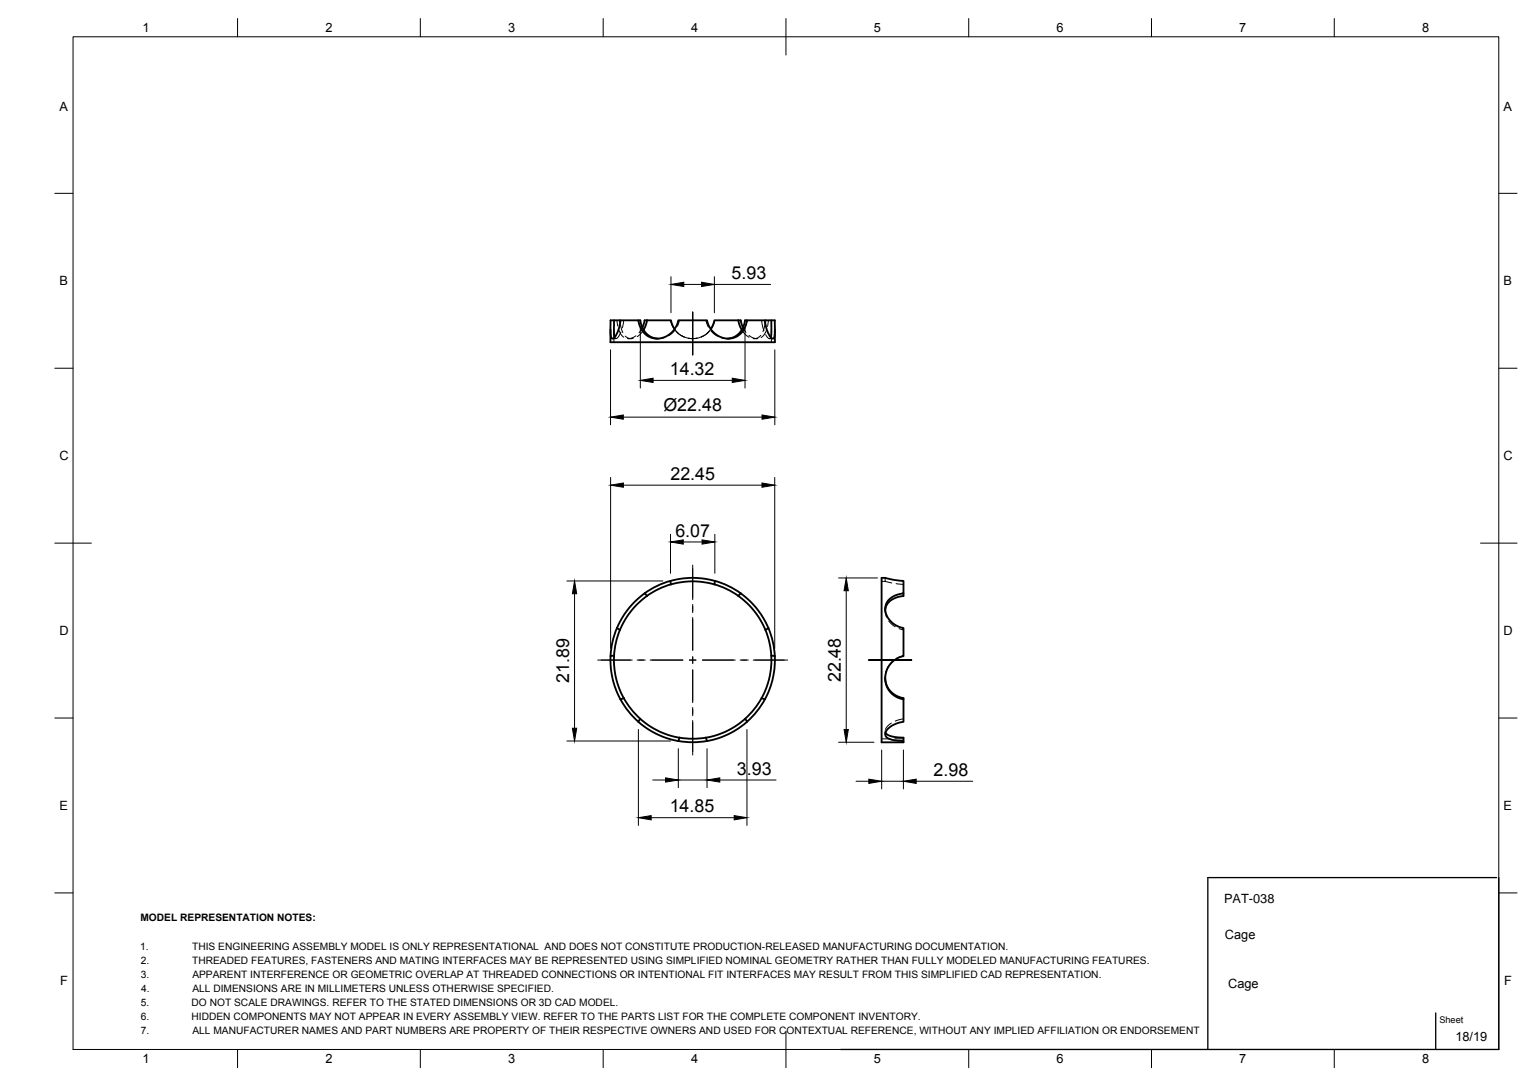
ISO-10303-21;
HEADER;
/* Generated by software containing ST-Developer
 * from STEP Tools, Inc. (www.steptools.com) 
 */

FILE_DESCRIPTION(
/* description */ ('Fork-mounted skate wheel'),
/* implementation_level */ '2;1');

FILE_NAME(
/* name */ 'Cage.step',
/* time_stamp */ '2026-10-29T16:11:26-07:00',
/* author */ (''),
/* organization */ (''),
/* preprocessor_version */ 'ST-DEVELOPER v20.2',
/* originating_system */ 'Autodesk Translation Framework v15.17.0.0',
/* authorisation */ '');

FILE_SCHEMA (('AUTOMOTIVE_DESIGN { 1 0 10303 214 3 1 1 }'));
ENDSEC;

DATA;
#10=MECHANICAL_DESIGN_GEOMETRIC_PRESENTATION_REPRESENTATION('',(#161),#3688);
#11=B_SPLINE_CURVE_WITH_KNOTS('',3,(#3211,#3212,#3213,#3214,#3215,#3216,
#3217,#3218,#3219,#3220,#3221,#3222,#3223,#3224,#3225,#3226,#3227,#3228,
#3229,#3230,#3231,#3232),.UNSPECIFIED.,.F.,.F.,(4,2,2,2,2,2,2,2,2,2,4),
(0.0591825211272536,0.157966726598481,0.236950089897721,0.315933453196962,
0.391576304923761,0.46721915665056,0.54286200837736,0.618504860104159,0.697488223403399,
0.77647158670264,0.875255792173867),.UNSPECIFIED.);
#12=B_SPLINE_CURVE_WITH_KNOTS('',3,(#3236,#3237,#3238,#3239,#3240,#3241,
#3242,#3243,#3244,#3245,#3246,#3247,#3248,#3249,#3250,#3251,#3252,#3253,
#3254,#3255,#3256,#3257),.UNSPECIFIED.,.F.,.F.,(4,2,2,2,2,2,2,2,2,2,4),
(0.0581119756758434,0.106553146291161,0.213106292582322,0.30849933801665,
0.386091982889075,0.4636846277615,0.541277272633925,0.61886991750635,0.714262962940678,
0.820816109231839,0.869257279847157),.UNSPECIFIED.);
#13=B_SPLINE_CURVE_WITH_KNOTS('',3,(#3263,#3264,#3265,#3266,#3267,#3268,
#3269,#3270,#3271,#3272,#3273,#3274,#3275,#3276,#3277,#3278,#3279,#3280,
#3281,#3282,#3283,#3284),.UNSPECIFIED.,.F.,.F.,(4,2,2,2,2,2,2,2,2,2,4),
(0.0581119756758434,0.106553146291161,0.213106292582322,0.30849933801665,
0.386091982889075,0.4636846277615,0.541277272633925,0.61886991750635,0.714262962940679,
0.820816109231839,0.869257279847157),.UNSPECIFIED.);
#14=B_SPLINE_CURVE_WITH_KNOTS('',3,(#3288,#3289,#3290,#3291,#3292,#3293,
#3294,#3295,#3296,#3297,#3298,#3299,#3300,#3301,#3302,#3303,#3304,#3305,
#3306,#3307,#3308,#3309),.UNSPECIFIED.,.F.,.F.,(4,2,2,2,2,2,2,2,2,2,4),
(0.0581119756758433,0.106553146291161,0.213106292582322,0.308499338016649,
0.386091982889075,0.4636846277615,0.541277272633925,0.61886991750635,0.714262962940678,
0.820816109231839,0.869257279847157),.UNSPECIFIED.);
#15=B_SPLINE_CURVE_WITH_KNOTS('',3,(#3318,#3319,#3320,#3321,#3322,#3323,
#3324,#3325,#3326,#3327,#3328,#3329,#3330,#3331,#3332,#3333,#3334,#3335,
#3336,#3337,#3338,#3339),.UNSPECIFIED.,.F.,.F.,(4,2,2,2,2,2,2,2,2,2,4),
(0.0581119756758433,0.106553146291161,0.213106292582322,0.30849933801665,
0.386091982889075,0.4636846277615,0.541277272633925,0.61886991750635,0.714262962940678,
0.820816109231839,0.869257279847157),.UNSPECIFIED.);
#16=B_SPLINE_CURVE_WITH_KNOTS('',3,(#3343,#3344,#3345,#3346,#3347,#3348,
#3349,#3350,#3351,#3352,#3353,#3354,#3355,#3356,#3357,#3358,#3359,#3360,
#3361,#3362,#3363,#3364),.UNSPECIFIED.,.F.,.F.,(4,2,2,2,2,2,2,2,2,2,4),
(0.0581119756758434,0.106553146291161,0.213106292582322,0.30849933801665,
0.386091982889075,0.4636846277615,0.541277272633925,0.61886991750635,0.714262962940678,
0.820816109231839,0.869257279847157),.UNSPECIFIED.);
#17=B_SPLINE_CURVE_WITH_KNOTS('',3,(#3368,#3369,#3370,#3371,#3372,#3373,
#3374,#3375,#3376,#3377,#3378,#3379,#3380,#3381,#3382,#3383,#3384,#3385,
#3386,#3387,#3388,#3389),.UNSPECIFIED.,.F.,.F.,(4,2,2,2,2,2,2,2,2,2,4),
(0.0581119756758434,0.106553146291161,0.213106292582322,0.30849933801665,
0.386091982889075,0.4636846277615,0.541277272633925,0.61886991750635,0.714262962940678,
0.820816109231839,0.869257279847157),.UNSPECIFIED.);
#18=B_SPLINE_CURVE_WITH_KNOTS('',3,(#3393,#3394,#3395,#3396,#3397,#3398,
#3399,#3400,#3401,#3402,#3403,#3404,#3405,#3406,#3407,#3408,#3409,#3410,
#3411,#3412,#3413,#3414),.UNSPECIFIED.,.F.,.F.,(4,2,2,2,2,2,2,2,2,2,4),
(0.0581119756758433,0.106553146291161,0.213106292582322,0.30849933801665,
0.386091982889075,0.4636846277615,0.541277272633925,0.61886991750635,0.714262962940678,
0.820816109231839,0.869257279847157),.UNSPECIFIED.);
#19=B_SPLINE_CURVE_WITH_KNOTS('',3,(#3422,#3423,#3424,#3425,#3426,#3427,
#3428,#3429,#3430,#3431,#3432,#3433,#3434,#3435,#3436,#3437,#3438,#3439,
#3440,#3441,#3442,#3443),.UNSPECIFIED.,.F.,.F.,(4,2,2,2,2,2,2,2,2,2,4),
(0.0591825211272536,0.157966726598481,0.236950089897721,0.315933453196962,
0.391576304923761,0.467219156650561,0.54286200837736,0.618504860104159,
0.697488223403399,0.77647158670264,0.875255792173867),.UNSPECIFIED.);
#20=B_SPLINE_CURVE_WITH_KNOTS('',3,(#3451,#3452,#3453,#3454,#3455,#3456,
#3457,#3458,#3459,#3460,#3461,#3462,#3463,#3464,#3465,#3466,#3467,#3468,
#3469,#3470,#3471,#3472),.UNSPECIFIED.,.F.,.F.,(4,2,2,2,2,2,2,2,2,2,4),
(0.0591825211272536,0.157966726598481,0.236950089897722,0.315933453196962,
0.391576304923761,0.467219156650561,0.54286200837736,0.618504860104159,
0.697488223403399,0.77647158670264,0.875255792173867),.UNSPECIFIED.);
#21=B_SPLINE_CURVE_WITH_KNOTS('',3,(#3482,#3483,#3484,#3485,#3486,#3487,
#3488,#3489,#3490,#3491,#3492,#3493,#3494,#3495,#3496,#3497,#3498,#3499,
#3500,#3501,#3502,#3503),.UNSPECIFIED.,.F.,.F.,(4,2,2,2,2,2,2,2,2,2,4),
(0.0591825211272536,0.157966726598481,0.236950089897721,0.315933453196962,
0.391576304923761,0.46721915665056,0.54286200837736,0.618504860104159,0.697488223403399,
0.77647158670264,0.875255792173867),.UNSPECIFIED.);
#22=B_SPLINE_CURVE_WITH_KNOTS('',3,(#3511,#3512,#3513,#3514,#3515,#3516,
#3517,#3518,#3519,#3520,#3521,#3522,#3523,#3524,#3525,#3526,#3527,#3528,
#3529,#3530,#3531,#3532),.UNSPECIFIED.,.F.,.F.,(4,2,2,2,2,2,2,2,2,2,4),
(0.0591825211272536,0.157966726598481,0.236950089897721,0.315933453196962,
0.391576304923761,0.46721915665056,0.542862008377359,0.618504860104159,
0.697488223403399,0.776471586702639,0.875255792173867),.UNSPECIFIED.);
#23=B_SPLINE_CURVE_WITH_KNOTS('',3,(#3540,#3541,#3542,#3543,#3544,#3545,
#3546,#3547,#3548,#3549,#3550,#3551,#3552,#3553,#3554,#3555,#3556,#3557,
#3558,#3559,#3560,#3561),.UNSPECIFIED.,.F.,.F.,(4,2,2,2,2,2,2,2,2,2,4),
(0.0591825211272536,0.157966726598481,0.236950089897721,0.315933453196962,
0.391576304923761,0.46721915665056,0.54286200837736,0.618504860104159,0.697488223403399,
0.77647158670264,0.875255792173867),.UNSPECIFIED.);
#24=B_SPLINE_CURVE_WITH_KNOTS('',3,(#3570,#3571,#3572,#3573,#3574,#3575,
#3576,#3577,#3578,#3579,#3580,#3581,#3582,#3583,#3584,#3585,#3586,#3587,
#3588,#3589,#3590,#3591),.UNSPECIFIED.,.F.,.F.,(4,2,2,2,2,2,2,2,2,2,4),
(0.0591825211272536,0.157966726598481,0.236950089897721,0.315933453196962,
0.391576304923761,0.46721915665056,0.542862008377359,0.618504860104159,
0.697488223403399,0.776471586702639,0.875255792173867),.UNSPECIFIED.);
#32=SPHERICAL_SURFACE('',#2134,0.309556);
#33=SPHERICAL_SURFACE('',#2150,0.309556);
#34=SPHERICAL_SURFACE('',#2155,0.309556);
#35=SPHERICAL_SURFACE('',#2161,0.309556);
#36=SPHERICAL_SURFACE('',#2166,0.309556);
#37=SPHERICAL_SURFACE('',#2171,0.309556);
#38=SPHERICAL_SURFACE('',#2179,0.309556);
#131=SHAPE_REPRESENTATION_RELATIONSHIP('SRR','None',#3756,#143);
#143=ADVANCED_BREP_SHAPE_REPRESENTATION('',(#179),#3685);
#161=STYLED_ITEM('',(#3896),#179);
#179=MANIFOLD_SOLID_BREP('Continuous crown cage',#1823);
#212=FACE_BOUND('',#518,.T.);
#262=PLANE('',#2147);
#263=PLANE('',#2152);
#264=PLANE('',#2157);
#265=PLANE('',#2163);
#266=PLANE('',#2168);
#267=PLANE('',#2177);
#268=PLANE('',#2181);
#269=PLANE('',#2182);
#360=FACE_OUTER_BOUND('',#502,.T.);
#361=FACE_OUTER_BOUND('',#503,.T.);
#362=FACE_OUTER_BOUND('',#504,.T.);
#363=FACE_OUTER_BOUND('',#505,.T.);
#364=FACE_OUTER_BOUND('',#506,.T.);
#365=FACE_OUTER_BOUND('',#507,.T.);
#366=FACE_OUTER_BOUND('',#508,.T.);
#367=FACE_OUTER_BOUND('',#509,.T.);
#368=FACE_OUTER_BOUND('',#510,.T.);
#369=FACE_OUTER_BOUND('',#511,.T.);
#370=FACE_OUTER_BOUND('',#512,.T.);
#371=FACE_OUTER_BOUND('',#513,.T.);
#372=FACE_OUTER_BOUND('',#514,.T.);
#373=FACE_OUTER_BOUND('',#515,.T.);
#374=FACE_OUTER_BOUND('',#516,.T.);
#375=FACE_OUTER_BOUND('',#517,.T.);
#376=FACE_OUTER_BOUND('',#519,.T.);
#502=EDGE_LOOP('',(#1529,#1530,#1531,#1532));
#503=EDGE_LOOP('',(#1533,#1534,#1535,#1536,#1537,#1538,#1539,#1540,#1541,
#1542,#1543,#1544,#1545,#1546,#1547,#1548,#1549,#1550));
#504=EDGE_LOOP('',(#1551,#1552,#1553,#1554));
#505=EDGE_LOOP('',(#1555,#1556,#1557,#1558));
#506=EDGE_LOOP('',(#1559,#1560,#1561,#1562));
#507=EDGE_LOOP('',(#1563,#1564,#1565,#1566));
#508=EDGE_LOOP('',(#1567,#1568,#1569,#1570,#1571,#1572));
#509=EDGE_LOOP('',(#1573,#1574,#1575,#1576));
#510=EDGE_LOOP('',(#1577,#1578,#1579,#1580));
#511=EDGE_LOOP('',(#1581,#1582,#1583,#1584));
#512=EDGE_LOOP('',(#1585,#1586,#1587,#1588));
#513=EDGE_LOOP('',(#1589,#1590,#1591,#1592));
#514=EDGE_LOOP('',(#1593,#1594,#1595,#1596,#1597,#1598,#1599,#1600,#1601,
#1602,#1603,#1604,#1605,#1606,#1607,#1608,#1609,#1610));
#515=EDGE_LOOP('',(#1611,#1612,#1613,#1614));
#516=EDGE_LOOP('',(#1615,#1616,#1617,#1618));
#517=EDGE_LOOP('',(#1619));
#518=EDGE_LOOP('',(#1620));
#519=EDGE_LOOP('',(#1621,#1622,#1623,#1624));
#624=LINE('',#3313,#718);
#625=LINE('',#3566,#719);
#718=VECTOR('',#2669,1.123812);
#719=VECTOR('',#2738,1.076188);
#796=CIRCLE('',#2135,0.303778037777585);
#797=CIRCLE('',#2136,0.303778037777585);
#798=CIRCLE('',#2138,1.123812);
#799=CIRCLE('',#2139,1.123812);
#800=CIRCLE('',#2140,1.123812);
#801=CIRCLE('',#2141,1.123812);
#802=CIRCLE('',#2142,1.123812);
#803=CIRCLE('',#2143,1.123812);
#804=CIRCLE('',#2144,1.123812);
#805=CIRCLE('',#2145,1.123812);
#806=CIRCLE('',#2146,1.123812);
#807=CIRCLE('',#2148,1.076188);
#808=CIRCLE('',#2149,0.303778037777585);
#809=CIRCLE('',#2151,0.303778037777585);
#810=CIRCLE('',#2153,1.076188);
#811=CIRCLE('',#2154,0.303778037777585);
#812=CIRCLE('',#2156,0.303778037777585);
#813=CIRCLE('',#2158,1.076188);
#814=CIRCLE('',#2159,1.076188);
#815=CIRCLE('',#2160,0.303778037777585);
#816=CIRCLE('',#2162,0.303778037777585);
#817=CIRCLE('',#2164,1.076188);
#818=CIRCLE('',#2165,0.303778037777585);
#819=CIRCLE('',#2167,0.303778037777585);
#820=CIRCLE('',#2169,1.076188);
#821=CIRCLE('',#2170,0.303778037777585);
#822=CIRCLE('',#2172,0.303778037777585);
#823=CIRCLE('',#2174,1.076188);
#824=CIRCLE('',#2175,1.076188);
#825=CIRCLE('',#2176,1.076188);
#826=CIRCLE('',#2178,0.303778037777585);
#827=CIRCLE('',#2180,0.303778037777585);
#951=VERTEX_POINT('',#3209);
#952=VERTEX_POINT('',#3210);
#953=VERTEX_POINT('',#3233);
#954=VERTEX_POINT('',#3235);
#955=VERTEX_POINT('',#3260);
#956=VERTEX_POINT('',#3262);
#957=VERTEX_POINT('',#3285);
#958=VERTEX_POINT('',#3287);
#959=VERTEX_POINT('',#3310);
#960=VERTEX_POINT('',#3312);
#961=VERTEX_POINT('',#3315);
#962=VERTEX_POINT('',#3317);
#963=VERTEX_POINT('',#3340);
#964=VERTEX_POINT('',#3342);
#965=VERTEX_POINT('',#3365);
#966=VERTEX_POINT('',#3367);
#967=VERTEX_POINT('',#3390);
#968=VERTEX_POINT('',#3392);
#969=VERTEX_POINT('',#3417);
#970=VERTEX_POINT('',#3421);
#971=VERTEX_POINT('',#3446);
#972=VERTEX_POINT('',#3450);
#973=VERTEX_POINT('',#3475);
#974=VERTEX_POINT('',#3477);
#975=VERTEX_POINT('',#3481);
#976=VERTEX_POINT('',#3506);
#977=VERTEX_POINT('',#3510);
#978=VERTEX_POINT('',#3535);
#979=VERTEX_POINT('',#3539);
#980=VERTEX_POINT('',#3564);
#981=VERTEX_POINT('',#3567);
#982=VERTEX_POINT('',#3569);
#1151=EDGE_CURVE('',#951,#952,#11,.T.);
#1152=EDGE_CURVE('',#953,#951,#796,.T.);
#1153=EDGE_CURVE('',#954,#953,#12,.T.);
#1154=EDGE_CURVE('',#952,#954,#797,.T.);
#1155=EDGE_CURVE('',#955,#953,#798,.T.);
#1156=EDGE_CURVE('',#955,#956,#13,.T.);
#1157=EDGE_CURVE('',#957,#956,#799,.T.);
#1158=EDGE_CURVE('',#957,#958,#14,.T.);
#1159=EDGE_CURVE('',#959,#958,#800,.T.);
#1160=EDGE_CURVE('',#959,#960,#624,.T.);
#1161=EDGE_CURVE('',#960,#960,#801,.T.);
#1162=EDGE_CURVE('',#961,#959,#802,.T.);
#1163=EDGE_CURVE('',#961,#962,#15,.T.);
#1164=EDGE_CURVE('',#963,#962,#803,.T.);
#1165=EDGE_CURVE('',#963,#964,#16,.T.);
#1166=EDGE_CURVE('',#965,#964,#804,.T.);
#1167=EDGE_CURVE('',#965,#966,#17,.T.);
#1168=EDGE_CURVE('',#967,#966,#805,.T.);
#1169=EDGE_CURVE('',#967,#968,#18,.T.);
#1170=EDGE_CURVE('',#954,#968,#806,.T.);
#1171=EDGE_CURVE('',#951,#969,#807,.T.);
#1172=EDGE_CURVE('',#969,#955,#808,.T.);
#1173=EDGE_CURVE('',#970,#969,#19,.T.);
#1174=EDGE_CURVE('',#956,#970,#809,.T.);
#1175=EDGE_CURVE('',#970,#971,#810,.T.);
#1176=EDGE_CURVE('',#971,#957,#811,.T.);
#1177=EDGE_CURVE('',#972,#971,#20,.T.);
#1178=EDGE_CURVE('',#958,#972,#812,.T.);
#1179=EDGE_CURVE('',#972,#973,#813,.T.);
#1180=EDGE_CURVE('',#973,#974,#814,.T.);
#1181=EDGE_CURVE('',#974,#961,#815,.T.);
#1182=EDGE_CURVE('',#975,#974,#21,.T.);
#1183=EDGE_CURVE('',#962,#975,#816,.T.);
#1184=EDGE_CURVE('',#975,#976,#817,.T.);
#1185=EDGE_CURVE('',#976,#963,#818,.T.);
#1186=EDGE_CURVE('',#977,#976,#22,.T.);
#1187=EDGE_CURVE('',#964,#977,#819,.T.);
#1188=EDGE_CURVE('',#977,#978,#820,.T.);
#1189=EDGE_CURVE('',#978,#965,#821,.T.);
#1190=EDGE_CURVE('',#979,#978,#23,.T.);
#1191=EDGE_CURVE('',#966,#979,#822,.T.);
#1192=EDGE_CURVE('',#980,#980,#823,.T.);
#1193=EDGE_CURVE('',#980,#973,#625,.T.);
#1194=EDGE_CURVE('',#981,#952,#824,.T.);
#1195=EDGE_CURVE('',#981,#982,#24,.T.);
#1196=EDGE_CURVE('',#979,#982,#825,.T.);
#1197=EDGE_CURVE('',#968,#981,#826,.T.);
#1198=EDGE_CURVE('',#982,#967,#827,.T.);
#1529=ORIENTED_EDGE('',*,*,#1151,.F.);
#1530=ORIENTED_EDGE('',*,*,#1152,.F.);
#1531=ORIENTED_EDGE('',*,*,#1153,.F.);
#1532=ORIENTED_EDGE('',*,*,#1154,.F.);
#1533=ORIENTED_EDGE('',*,*,#1153,.T.);
#1534=ORIENTED_EDGE('',*,*,#1155,.F.);
#1535=ORIENTED_EDGE('',*,*,#1156,.T.);
#1536=ORIENTED_EDGE('',*,*,#1157,.F.);
#1537=ORIENTED_EDGE('',*,*,#1158,.T.);
#1538=ORIENTED_EDGE('',*,*,#1159,.F.);
#1539=ORIENTED_EDGE('',*,*,#1160,.T.);
#1540=ORIENTED_EDGE('',*,*,#1161,.F.);
#1541=ORIENTED_EDGE('',*,*,#1160,.F.);
#1542=ORIENTED_EDGE('',*,*,#1162,.F.);
#1543=ORIENTED_EDGE('',*,*,#1163,.T.);
#1544=ORIENTED_EDGE('',*,*,#1164,.F.);
#1545=ORIENTED_EDGE('',*,*,#1165,.T.);
#1546=ORIENTED_EDGE('',*,*,#1166,.F.);
#1547=ORIENTED_EDGE('',*,*,#1167,.T.);
#1548=ORIENTED_EDGE('',*,*,#1168,.F.);
#1549=ORIENTED_EDGE('',*,*,#1169,.T.);
#1550=ORIENTED_EDGE('',*,*,#1170,.F.);
#1551=ORIENTED_EDGE('',*,*,#1152,.T.);
#1552=ORIENTED_EDGE('',*,*,#1171,.T.);
#1553=ORIENTED_EDGE('',*,*,#1172,.T.);
#1554=ORIENTED_EDGE('',*,*,#1155,.T.);
#1555=ORIENTED_EDGE('',*,*,#1173,.F.);
#1556=ORIENTED_EDGE('',*,*,#1174,.F.);
#1557=ORIENTED_EDGE('',*,*,#1156,.F.);
#1558=ORIENTED_EDGE('',*,*,#1172,.F.);
#1559=ORIENTED_EDGE('',*,*,#1174,.T.);
#1560=ORIENTED_EDGE('',*,*,#1175,.T.);
#1561=ORIENTED_EDGE('',*,*,#1176,.T.);
#1562=ORIENTED_EDGE('',*,*,#1157,.T.);
#1563=ORIENTED_EDGE('',*,*,#1177,.F.);
#1564=ORIENTED_EDGE('',*,*,#1178,.F.);
#1565=ORIENTED_EDGE('',*,*,#1158,.F.);
#1566=ORIENTED_EDGE('',*,*,#1176,.F.);
#1567=ORIENTED_EDGE('',*,*,#1178,.T.);
#1568=ORIENTED_EDGE('',*,*,#1179,.T.);
#1569=ORIENTED_EDGE('',*,*,#1180,.T.);
#1570=ORIENTED_EDGE('',*,*,#1181,.T.);
#1571=ORIENTED_EDGE('',*,*,#1162,.T.);
#1572=ORIENTED_EDGE('',*,*,#1159,.T.);
#1573=ORIENTED_EDGE('',*,*,#1182,.F.);
#1574=ORIENTED_EDGE('',*,*,#1183,.F.);
#1575=ORIENTED_EDGE('',*,*,#1163,.F.);
#1576=ORIENTED_EDGE('',*,*,#1181,.F.);
#1577=ORIENTED_EDGE('',*,*,#1183,.T.);
#1578=ORIENTED_EDGE('',*,*,#1184,.T.);
#1579=ORIENTED_EDGE('',*,*,#1185,.T.);
#1580=ORIENTED_EDGE('',*,*,#1164,.T.);
#1581=ORIENTED_EDGE('',*,*,#1186,.F.);
#1582=ORIENTED_EDGE('',*,*,#1187,.F.);
#1583=ORIENTED_EDGE('',*,*,#1165,.F.);
#1584=ORIENTED_EDGE('',*,*,#1185,.F.);
#1585=ORIENTED_EDGE('',*,*,#1187,.T.);
#1586=ORIENTED_EDGE('',*,*,#1188,.T.);
#1587=ORIENTED_EDGE('',*,*,#1189,.T.);
#1588=ORIENTED_EDGE('',*,*,#1166,.T.);
#1589=ORIENTED_EDGE('',*,*,#1167,.F.);
#1590=ORIENTED_EDGE('',*,*,#1189,.F.);
#1591=ORIENTED_EDGE('',*,*,#1190,.F.);
#1592=ORIENTED_EDGE('',*,*,#1191,.F.);
#1593=ORIENTED_EDGE('',*,*,#1192,.F.);
#1594=ORIENTED_EDGE('',*,*,#1193,.T.);
#1595=ORIENTED_EDGE('',*,*,#1179,.F.);
#1596=ORIENTED_EDGE('',*,*,#1177,.T.);
#1597=ORIENTED_EDGE('',*,*,#1175,.F.);
#1598=ORIENTED_EDGE('',*,*,#1173,.T.);
#1599=ORIENTED_EDGE('',*,*,#1171,.F.);
#1600=ORIENTED_EDGE('',*,*,#1151,.T.);
#1601=ORIENTED_EDGE('',*,*,#1194,.F.);
#1602=ORIENTED_EDGE('',*,*,#1195,.T.);
#1603=ORIENTED_EDGE('',*,*,#1196,.F.);
#1604=ORIENTED_EDGE('',*,*,#1190,.T.);
#1605=ORIENTED_EDGE('',*,*,#1188,.F.);
#1606=ORIENTED_EDGE('',*,*,#1186,.T.);
#1607=ORIENTED_EDGE('',*,*,#1184,.F.);
#1608=ORIENTED_EDGE('',*,*,#1182,.T.);
#1609=ORIENTED_EDGE('',*,*,#1180,.F.);
#1610=ORIENTED_EDGE('',*,*,#1193,.F.);
#1611=ORIENTED_EDGE('',*,*,#1154,.T.);
#1612=ORIENTED_EDGE('',*,*,#1170,.T.);
#1613=ORIENTED_EDGE('',*,*,#1197,.T.);
#1614=ORIENTED_EDGE('',*,*,#1194,.T.);
#1615=ORIENTED_EDGE('',*,*,#1169,.F.);
#1616=ORIENTED_EDGE('',*,*,#1198,.F.);
#1617=ORIENTED_EDGE('',*,*,#1195,.F.);
#1618=ORIENTED_EDGE('',*,*,#1197,.F.);
#1619=ORIENTED_EDGE('',*,*,#1161,.T.);
#1620=ORIENTED_EDGE('',*,*,#1192,.T.);
#1621=ORIENTED_EDGE('',*,*,#1191,.T.);
#1622=ORIENTED_EDGE('',*,*,#1196,.T.);
#1623=ORIENTED_EDGE('',*,*,#1198,.T.);
#1624=ORIENTED_EDGE('',*,*,#1168,.T.);
#1686=CYLINDRICAL_SURFACE('',#2137,1.123812);
#1687=CYLINDRICAL_SURFACE('',#2173,1.076188);
#1778=ADVANCED_FACE('',(#360),#32,.F.);
#1779=ADVANCED_FACE('',(#361),#1686,.T.);
#1780=ADVANCED_FACE('',(#362),#262,.T.);
#1781=ADVANCED_FACE('',(#363),#33,.F.);
#1782=ADVANCED_FACE('',(#364),#263,.T.);
#1783=ADVANCED_FACE('',(#365),#34,.F.);
#1784=ADVANCED_FACE('',(#366),#264,.T.);
#1785=ADVANCED_FACE('',(#367),#35,.F.);
#1786=ADVANCED_FACE('',(#368),#265,.T.);
#1787=ADVANCED_FACE('',(#369),#36,.F.);
#1788=ADVANCED_FACE('',(#370),#266,.T.);
#1789=ADVANCED_FACE('',(#371),#37,.F.);
#1790=ADVANCED_FACE('',(#372),#1687,.F.);
#1791=ADVANCED_FACE('',(#373),#267,.T.);
#1792=ADVANCED_FACE('',(#374),#38,.F.);
#1793=ADVANCED_FACE('',(#375,#212),#268,.T.);
#1794=ADVANCED_FACE('',(#376),#269,.T.);
#1823=CLOSED_SHELL('',(#1778,#1779,#1780,#1781,#1782,#1783,#1784,#1785,
#1786,#1787,#1788,#1789,#1790,#1791,#1792,#1793,#1794));
#2133=AXIS2_PLACEMENT_3D('',#3207,#2653,#2654);
#2134=AXIS2_PLACEMENT_3D('',#3208,#2655,#2656);
#2135=AXIS2_PLACEMENT_3D('',#3234,#2657,#2658);
#2136=AXIS2_PLACEMENT_3D('',#3258,#2659,#2660);
#2137=AXIS2_PLACEMENT_3D('',#3259,#2661,#2662);
#2138=AXIS2_PLACEMENT_3D('',#3261,#2663,#2664);
#2139=AXIS2_PLACEMENT_3D('',#3286,#2665,#2666);
#2140=AXIS2_PLACEMENT_3D('',#3311,#2667,#2668);
#2141=AXIS2_PLACEMENT_3D('',#3314,#2670,#2671);
#2142=AXIS2_PLACEMENT_3D('',#3316,#2672,#2673);
#2143=AXIS2_PLACEMENT_3D('',#3341,#2674,#2675);
#2144=AXIS2_PLACEMENT_3D('',#3366,#2676,#2677);
#2145=AXIS2_PLACEMENT_3D('',#3391,#2678,#2679);
#2146=AXIS2_PLACEMENT_3D('',#3415,#2680,#2681);
#2147=AXIS2_PLACEMENT_3D('',#3416,#2682,#2683);
#2148=AXIS2_PLACEMENT_3D('',#3418,#2684,#2685);
#2149=AXIS2_PLACEMENT_3D('',#3419,#2686,#2687);
#2150=AXIS2_PLACEMENT_3D('',#3420,#2688,#2689);
#2151=AXIS2_PLACEMENT_3D('',#3444,#2690,#2691);
#2152=AXIS2_PLACEMENT_3D('',#3445,#2692,#2693);
#2153=AXIS2_PLACEMENT_3D('',#3447,#2694,#2695);
#2154=AXIS2_PLACEMENT_3D('',#3448,#2696,#2697);
#2155=AXIS2_PLACEMENT_3D('',#3449,#2698,#2699);
#2156=AXIS2_PLACEMENT_3D('',#3473,#2700,#2701);
#2157=AXIS2_PLACEMENT_3D('',#3474,#2702,#2703);
#2158=AXIS2_PLACEMENT_3D('',#3476,#2704,#2705);
#2159=AXIS2_PLACEMENT_3D('',#3478,#2706,#2707);
#2160=AXIS2_PLACEMENT_3D('',#3479,#2708,#2709);
#2161=AXIS2_PLACEMENT_3D('',#3480,#2710,#2711);
#2162=AXIS2_PLACEMENT_3D('',#3504,#2712,#2713);
#2163=AXIS2_PLACEMENT_3D('',#3505,#2714,#2715);
#2164=AXIS2_PLACEMENT_3D('',#3507,#2716,#2717);
#2165=AXIS2_PLACEMENT_3D('',#3508,#2718,#2719);
#2166=AXIS2_PLACEMENT_3D('',#3509,#2720,#2721);
#2167=AXIS2_PLACEMENT_3D('',#3533,#2722,#2723);
#2168=AXIS2_PLACEMENT_3D('',#3534,#2724,#2725);
#2169=AXIS2_PLACEMENT_3D('',#3536,#2726,#2727);
#2170=AXIS2_PLACEMENT_3D('',#3537,#2728,#2729);
#2171=AXIS2_PLACEMENT_3D('',#3538,#2730,#2731);
#2172=AXIS2_PLACEMENT_3D('',#3562,#2732,#2733);
#2173=AXIS2_PLACEMENT_3D('',#3563,#2734,#2735);
#2174=AXIS2_PLACEMENT_3D('',#3565,#2736,#2737);
#2175=AXIS2_PLACEMENT_3D('',#3568,#2739,#2740);
#2176=AXIS2_PLACEMENT_3D('',#3592,#2741,#2742);
#2177=AXIS2_PLACEMENT_3D('',#3593,#2743,#2744);
#2178=AXIS2_PLACEMENT_3D('',#3594,#2745,#2746);
#2179=AXIS2_PLACEMENT_3D('',#3595,#2747,#2748);
#2180=AXIS2_PLACEMENT_3D('',#3596,#2749,#2750);
#2181=AXIS2_PLACEMENT_3D('',#3597,#2751,#2752);
#2182=AXIS2_PLACEMENT_3D('',#3598,#2753,#2754);
#2653=DIRECTION('axis',(0.,0.,1.));
#2654=DIRECTION('refdir',(1.,0.,0.));
#2655=DIRECTION('center_axis',(0.,0.,1.));
#2656=DIRECTION('ref_axis',(1.,0.,0.));
#2657=DIRECTION('center_axis',(0.,-1.,0.));
#2658=DIRECTION('ref_axis',(0.,0.,-1.));
#2659=DIRECTION('center_axis',(0.,-1.,0.));
#2660=DIRECTION('ref_axis',(0.,0.,-1.));
#2661=DIRECTION('center_axis',(0.,1.,0.));
#2662=DIRECTION('ref_axis',(1.,0.,0.));
#2663=DIRECTION('center_axis',(0.,1.,0.));
#2664=DIRECTION('ref_axis',(1.,0.,0.));
#2665=DIRECTION('center_axis',(0.,1.,0.));
#2666=DIRECTION('ref_axis',(1.,0.,0.));
#2667=DIRECTION('center_axis',(0.,1.,0.));
#2668=DIRECTION('ref_axis',(1.,0.,0.));
#2669=DIRECTION('',(0.,-1.,0.));
#2670=DIRECTION('center_axis',(0.,-1.,0.));
#2671=DIRECTION('ref_axis',(1.,0.,0.));
#2672=DIRECTION('center_axis',(0.,1.,0.));
#2673=DIRECTION('ref_axis',(1.,0.,0.));
#2674=DIRECTION('center_axis',(0.,1.,0.));
#2675=DIRECTION('ref_axis',(1.,0.,0.));
#2676=DIRECTION('center_axis',(0.,1.,0.));
#2677=DIRECTION('ref_axis',(1.,0.,0.));
#2678=DIRECTION('center_axis',(0.,1.,0.));
#2679=DIRECTION('ref_axis',(1.,0.,0.));
#2680=DIRECTION('center_axis',(0.,1.,0.));
#2681=DIRECTION('ref_axis',(1.,0.,0.));
#2682=DIRECTION('center_axis',(0.,1.,0.));
#2683=DIRECTION('ref_axis',(1.,0.,0.));
#2684=DIRECTION('center_axis',(0.,-1.,0.));
#2685=DIRECTION('ref_axis',(1.,0.,0.));
#2686=DIRECTION('center_axis',(0.,-1.,0.));
#2687=DIRECTION('ref_axis',(0.,0.,-1.));
#2688=DIRECTION('center_axis',(8.96625347776458E-17,0.,1.));
#2689=DIRECTION('ref_axis',(1.,0.,0.));
#2690=DIRECTION('center_axis',(0.,-1.,0.));
#2691=DIRECTION('ref_axis',(0.,0.,-1.));
#2692=DIRECTION('center_axis',(0.,1.,0.));
#2693=DIRECTION('ref_axis',(1.,0.,0.));
#2694=DIRECTION('center_axis',(0.,-1.,0.));
#2695=DIRECTION('ref_axis',(1.,0.,0.));
#2696=DIRECTION('center_axis',(0.,-1.,0.));
#2697=DIRECTION('ref_axis',(0.,0.,-1.));
#2698=DIRECTION('center_axis',(0.,0.,1.));
#2699=DIRECTION('ref_axis',(1.,0.,0.));
#2700=DIRECTION('center_axis',(0.,-1.,0.));
#2701=DIRECTION('ref_axis',(0.,0.,-1.));
#2702=DIRECTION('center_axis',(0.,1.,0.));
#2703=DIRECTION('ref_axis',(1.,0.,0.));
#2704=DIRECTION('center_axis',(0.,-1.,0.));
#2705=DIRECTION('ref_axis',(1.,0.,0.));
#2706=DIRECTION('center_axis',(0.,-1.,0.));
#2707=DIRECTION('ref_axis',(1.,0.,0.));
#2708=DIRECTION('center_axis',(0.,-1.,0.));
#2709=DIRECTION('ref_axis',(0.,0.,-1.));
#2710=DIRECTION('center_axis',(0.,0.,1.));
#2711=DIRECTION('ref_axis',(1.,0.,0.));
#2712=DIRECTION('center_axis',(0.,-1.,0.));
#2713=DIRECTION('ref_axis',(0.,0.,-1.));
#2714=DIRECTION('center_axis',(0.,1.,0.));
#2715=DIRECTION('ref_axis',(1.,0.,0.));
#2716=DIRECTION('center_axis',(0.,-1.,0.));
#2717=DIRECTION('ref_axis',(1.,0.,0.));
#2718=DIRECTION('center_axis',(0.,-1.,0.));
#2719=DIRECTION('ref_axis',(0.,0.,-1.));
#2720=DIRECTION('center_axis',(8.96625347776458E-17,0.,1.));
#2721=DIRECTION('ref_axis',(1.,0.,0.));
#2722=DIRECTION('center_axis',(0.,-1.,0.));
#2723=DIRECTION('ref_axis',(0.,0.,-1.));
#2724=DIRECTION('center_axis',(0.,1.,0.));
#2725=DIRECTION('ref_axis',(1.,0.,0.));
#2726=DIRECTION('center_axis',(0.,-1.,0.));
#2727=DIRECTION('ref_axis',(1.,0.,0.));
#2728=DIRECTION('center_axis',(0.,-1.,0.));
#2729=DIRECTION('ref_axis',(0.,0.,-1.));
#2730=DIRECTION('center_axis',(0.,0.,1.));
#2731=DIRECTION('ref_axis',(1.,0.,0.));
#2732=DIRECTION('center_axis',(0.,-1.,0.));
#2733=DIRECTION('ref_axis',(0.,0.,-1.));
#2734=DIRECTION('center_axis',(0.,1.,0.));
#2735=DIRECTION('ref_axis',(1.,0.,0.));
#2736=DIRECTION('center_axis',(0.,1.,0.));
#2737=DIRECTION('ref_axis',(1.,0.,0.));
#2738=DIRECTION('',(0.,1.,0.));
#2739=DIRECTION('center_axis',(0.,-1.,0.));
#2740=DIRECTION('ref_axis',(1.,0.,0.));
#2741=DIRECTION('center_axis',(0.,-1.,0.));
#2742=DIRECTION('ref_axis',(1.,0.,0.));
#2743=DIRECTION('center_axis',(0.,1.,0.));
#2744=DIRECTION('ref_axis',(1.,0.,0.));
#2745=DIRECTION('center_axis',(0.,-1.,0.));
#2746=DIRECTION('ref_axis',(0.,0.,-1.));
#2747=DIRECTION('center_axis',(0.,0.,1.));
#2748=DIRECTION('ref_axis',(1.,0.,0.));
#2749=DIRECTION('center_axis',(0.,-1.,0.));
#2750=DIRECTION('ref_axis',(0.,0.,-1.));
#2751=DIRECTION('center_axis',(0.,-1.,0.));
#2752=DIRECTION('ref_axis',(-1.,0.,0.));
#2753=DIRECTION('center_axis',(0.,1.,0.));
#2754=DIRECTION('ref_axis',(1.,0.,0.));
#3207=CARTESIAN_POINT('',(0.,0.,0.));
#3208=CARTESIAN_POINT('Origin',(0.685838782044607,0.,0.860014630714833));
#3209=CARTESIAN_POINT('',(0.413083465285518,-0.05953,0.993751811093549));
#3210=CARTESIAN_POINT('',(0.876916659919095,-0.05953,0.623857181492959));
#3211=CARTESIAN_POINT('Ctrl Pts',(0.413083465285518,-0.05953,0.993751811093549));
#3212=CARTESIAN_POINT('Ctrl Pts',(0.419070565453383,-0.0925528133349865,
0.991263089003441));
#3213=CARTESIAN_POINT('Ctrl Pts',(0.430199341854858,-0.124911173756694,
0.986608710139579));
#3214=CARTESIAN_POINT('Ctrl Pts',(0.457978755888596,-0.177924977804098,
0.973971221090534));
#3215=CARTESIAN_POINT('Ctrl Pts',(0.473077587363685,-0.199697230012983,
0.966820759530997));
#3216=CARTESIAN_POINT('Ctrl Pts',(0.507057380724533,-0.237895043532788,
0.949440676105255));
#3217=CARTESIAN_POINT('Ctrl Pts',(0.525933334162555,-0.254319232363049,
0.939198248544428));
#3218=CARTESIAN_POINT('Ctrl Pts',(0.564362943424238,-0.28018331644634,0.916597376014514));
#3219=CARTESIAN_POINT('Ctrl Pts',(0.585840553788742,-0.29104845371857,0.903141581680914));
#3220=CARTESIAN_POINT('Ctrl Pts',(0.629305439856167,-0.30527573347708,0.873412008702649));
#3221=CARTESIAN_POINT('Ctrl Pts',(0.651278921914856,-0.308638795020976,
0.857118508332695));
#3222=CARTESIAN_POINT('Ctrl Pts',(0.690705563850638,-0.308638795020976,
0.825676810575914));
#3223=CARTESIAN_POINT('Ctrl Pts',(0.711480111898423,-0.30527573347708,0.807879894508811));
#3224=CARTESIAN_POINT('Ctrl Pts',(0.750136149454208,-0.29104845371857,0.772120216227122));
#3225=CARTESIAN_POINT('Ctrl Pts',(0.768033796848072,-0.28018331644634,0.754175290318038));
#3226=CARTESIAN_POINT('Ctrl Pts',(0.798619410861634,-0.254319232363049,
0.721738358858166));
#3227=CARTESIAN_POINT('Ctrl Pts',(0.812805334167529,-0.237895043532788,
0.705614819529209));
#3228=CARTESIAN_POINT('Ctrl Pts',(0.837310877969633,-0.199697230012983,
0.676354402927683));
#3229=CARTESIAN_POINT('Ctrl Pts',(0.847641868610495,-0.177924977804098,
0.663225258065736));
#3230=CARTESIAN_POINT('Ctrl Pts',(0.866144010579847,-0.124911173756694,
0.638954437806245));
#3231=CARTESIAN_POINT('Ctrl Pts',(0.873158080166742,-0.0925528133349865,
0.62914037979579));
#3232=CARTESIAN_POINT('Ctrl Pts',(0.876916659919095,-0.05953,0.623857181492959));
#3233=CARTESIAN_POINT('',(0.437601487681057,-0.05953,1.03511272300331));
#3234=CARTESIAN_POINT('Origin',(0.685838782044607,-0.05953,0.860014630714833));
#3235=CARTESIAN_POINT('',(0.911784794170997,-0.05953,0.656964154625313));
#3236=CARTESIAN_POINT('Ctrl Pts',(0.911784794170998,-0.0595300000000001,
0.656964154625312));
#3237=CARTESIAN_POINT('Ctrl Pts',(0.909827729890942,-0.0762225747374255,
0.659680317203144));
#3238=CARTESIAN_POINT('Ctrl Pts',(0.907004864562642,-0.0928409665394228,
0.663576540841106));
#3239=CARTESIAN_POINT('Ctrl Pts',(0.895234408667242,-0.144299303100741,
0.679480524217551));
#3240=CARTESIAN_POINT('Ctrl Pts',(0.882797231409153,-0.177024326825049,
0.695831250979106));
#3241=CARTESIAN_POINT('Ctrl Pts',(0.854332839576145,-0.227269801620064,
0.73042219438957));
#3242=CARTESIAN_POINT('Ctrl Pts',(0.834863020612702,-0.251265615809407,
0.752807465209441));
#3243=CARTESIAN_POINT('Ctrl Pts',(0.800439809856111,-0.279889827963178,
0.789147407129766));
#3244=CARTESIAN_POINT('Ctrl Pts',(0.781998747691871,-0.290879136862659,
0.80756613568454));
#3245=CARTESIAN_POINT('Ctrl Pts',(0.742239891936898,-0.305251990234487,
0.844254137480382));
#3246=CARTESIAN_POINT('Ctrl Pts',(0.720906778729541,-0.308638795020976,
0.862505527716294));
#3247=CARTESIAN_POINT('Ctrl Pts',(0.680463863683392,-0.308638795020976,
0.894757676234429));
#3248=CARTESIAN_POINT('Ctrl Pts',(0.657923009631182,-0.305251990234488,
0.91149460735272));
#3249=CARTESIAN_POINT('Ctrl Pts',(0.613307674922609,-0.290879136862659,
0.942092777160053));
#3250=CARTESIAN_POINT('Ctrl Pts',(0.591247219971725,-0.279889827963178,
0.955972930713954));
#3251=CARTESIAN_POINT('Ctrl Pts',(0.548158511259202,-0.251265615809407,
0.981446681891443));
#3252=CARTESIAN_POINT('Ctrl Pts',(0.522002043615455,-0.227269801620063,
0.995447160474328));
#3253=CARTESIAN_POINT('Ctrl Pts',(0.481944444320713,-0.177024326825049,
1.01550068154148));
#3254=CARTESIAN_POINT('Ctrl Pts',(0.463236132117164,-0.14429930310074,1.0239876538093));
#3255=CARTESIAN_POINT('Ctrl Pts',(0.445111721969657,-0.0928409665394226,
1.03192403056628));
#3256=CARTESIAN_POINT('Ctrl Pts',(0.440685038163619,-0.0762225747374254,
1.03380912944435));
#3257=CARTESIAN_POINT('Ctrl Pts',(0.437601487681056,-0.05953,1.03511272300331));
#3258=CARTESIAN_POINT('Origin',(0.685838782044607,-0.05953,0.860014630714833));
#3259=CARTESIAN_POINT('Origin',(0.,-0.208355,0.));
#3260=CARTESIAN_POINT('',(0.0548532617164168,-0.05953,1.12247250791415));
#3261=CARTESIAN_POINT('Origin',(0.,-0.05953,0.));
#3262=CARTESIAN_POINT('',(-0.536443649899848,-0.05953,0.987512846410683));
#3263=CARTESIAN_POINT('Ctrl Pts',(0.0548532617164173,-0.0595300000000001,
1.12247250791414));
#3264=CARTESIAN_POINT('Ctrl Pts',(0.05150947068137,-0.0762225747374254,
1.12263591311425));
#3265=CARTESIAN_POINT('Ctrl Pts',(0.0467032526342597,-0.0928409665394227,
1.12285816383385));
#3266=CARTESIAN_POINT('Ctrl Pts',(0.0269302585198975,-0.144299303100741,
1.12357162229597));
#3267=CARTESIAN_POINT('Ctrl Pts',(0.006392292392153,-0.177024326825049,
1.12404235695137));
#3268=CARTESIAN_POINT('Ctrl Pts',(-0.0383992541984087,-0.227269801620063,
1.12335509974011));
#3269=CARTESIAN_POINT('Ctrl Pts',(-0.0680399972366993,-0.251265615809407,
1.12208997038458));
#3270=CARTESIAN_POINT('Ctrl Pts',(-0.117914228755037,-0.279889827963178,
1.1178344036749));
#3271=CARTESIAN_POINT('Ctrl Pts',(-0.14381238480104,-0.290879136862659,
1.11490049012186));
#3272=CARTESIAN_POINT('Ctrl Pts',(-0.19728546073067,-0.305251990234488,
1.10669035995599));
#3273=CARTESIAN_POINT('Ctrl Pts',(-0.224855950742601,-0.308638795020976,
1.10139101611326));
#3274=CARTESIAN_POINT('Ctrl Pts',(-0.275287440920027,-0.308638795020976,
1.0898803575765));
#3275=CARTESIAN_POINT('Ctrl Pts',(-0.302426893214945,-0.305251990234488,
1.08269251410343));
#3276=CARTESIAN_POINT('Ctrl Pts',(-0.35416671187353,-0.290879136862659,
1.06688848765783));
#3277=CARTESIAN_POINT('Ctrl Pts',(-0.3787731215897,-0.279889827963178,1.05829506364875));
#3278=CARTESIAN_POINT('Ctrl Pts',(-0.425554672694338,-0.251265615809407,
1.04048957871266));
#3279=CARTESIAN_POINT('Ctrl Pts',(-0.452808978448581,-0.227269801620063,
1.02876878445619));
#3280=CARTESIAN_POINT('Ctrl Pts',(-0.493462957200432,-0.177024326825049,
1.0099536580922));
#3281=CARTESIAN_POINT('Ctrl Pts',(-0.511762781179148,-0.14429930310074,
1.00061845128527));
#3282=CARTESIAN_POINT('Ctrl Pts',(-0.529268075276157,-0.0928409665394226,
0.991396466802468));
#3283=CARTESIAN_POINT('Ctrl Pts',(-0.533501897135713,-0.0762225747374254,
0.989110885965947));
#3284=CARTESIAN_POINT('Ctrl Pts',(-0.536443649899848,-0.0595300000000001,
0.987512846410683));
#3285=CARTESIAN_POINT('',(-0.843383895613249,-0.05953,0.742736168477219));
#3286=CARTESIAN_POINT('Origin',(0.,-0.05953,0.));
#3287=CARTESIAN_POINT('',(-1.10653577764992,-0.05953,0.196295654879792));
#3288=CARTESIAN_POINT('Ctrl Pts',(-0.843383895613249,-0.0595300000000001,
0.742736168477219));
#3289=CARTESIAN_POINT('Ctrl Pts',(-0.84559647055299,-0.0762225747374255,
0.740223768851062));
#3290=CARTESIAN_POINT('Ctrl Pts',(-0.848766861100456,-0.0928409665394227,
0.736604687327351));
#3291=CARTESIAN_POINT('Ctrl Pts',(-0.861652925570091,-0.144299303100741,
0.721590372101268));
#3292=CARTESIAN_POINT('Ctrl Pts',(-0.87482617317514,-0.177024326825049,
0.705826641853758));
#3293=CARTESIAN_POINT('Ctrl Pts',(-0.902215926359523,-0.227269801620063,
0.670378702718353));
#3294=CARTESIAN_POINT('Ctrl Pts',(-0.919707509403859,-0.251265615809407,
0.646415841396062));
#3295=CARTESIAN_POINT('Ctrl Pts',(-0.947476448101718,-0.279889827963178,
0.604769294586516));
#3296=CARTESIAN_POINT('Ctrl Pts',(-0.961329858300736,-0.290879136862659,
0.582692035672022));
#3297=CARTESIAN_POINT('Ctrl Pts',(-0.988250837578047,-0.305251990234488,
0.535766169015486));
#3298=CARTESIAN_POINT('Ctrl Pts',(-1.00129756308006,-0.308638795020976,
0.510906605094603));
#3299=CARTESIAN_POINT('Ctrl Pts',(-1.02374168767024,-0.308638795020976,
0.46430090015576));
#3300=CARTESIAN_POINT('Ctrl Pts',(-1.03504317708586,-0.305251990234488,
0.438600874831839));
#3301=CARTESIAN_POINT('Ctrl Pts',(-1.05494634094458,-0.290879136862659,
0.388295406390235));
#3302=CARTESIAN_POINT('Ctrl Pts',(-1.06356957703048,-0.279889827963178,
0.363699428370917));
#3303=CARTESIAN_POINT('Ctrl Pts',(-1.0788165083757,-0.251265615809407,0.316022600643821));
#3304=CARTESIAN_POINT('Ctrl Pts',(-1.08664560412098,-0.227269801620063,
0.287406530683752));
#3305=CARTESIAN_POINT('Ctrl Pts',(-1.09728268713976,-0.177024326825049,
0.243890930799337));
#3306=CARTESIAN_POINT('Ctrl Pts',(-1.10139388218929,-0.144299303100741,
0.22376314604679));
#3307=CARTESIAN_POINT('Ctrl Pts',(-1.10509821673782,-0.0928409665394227,
0.204327142733961));
#3308=CARTESIAN_POINT('Ctrl Pts',(-1.10595102243643,-0.0762225747374254,
0.199591971170104));
#3309=CARTESIAN_POINT('Ctrl Pts',(-1.10653577764992,-0.0595300000000001,
0.196295654879792));
#3310=CARTESIAN_POINT('',(-1.123812,-0.05953,1.37627276864339E-16));
#3311=CARTESIAN_POINT('Origin',(0.,-0.05953,0.));
#3312=CARTESIAN_POINT('',(-1.123812,-0.35718,1.37627276864339E-16));
#3313=CARTESIAN_POINT('',(-1.123812,-0.208355,1.37627276864339E-16));
#3314=CARTESIAN_POINT('Origin',(0.,-0.35718,0.));
#3315=CARTESIAN_POINT('',(-1.10653577764992,-0.05953,-0.196295654879793));
#3316=CARTESIAN_POINT('Origin',(0.,-0.05953,0.));
#3317=CARTESIAN_POINT('',(-0.843383895613249,-0.05953,-0.742736168477219));
#3318=CARTESIAN_POINT('Ctrl Pts',(-1.10653577764992,-0.0595300000000001,
-0.196295654879792));
#3319=CARTESIAN_POINT('Ctrl Pts',(-1.10595102243643,-0.0762225747374255,
-0.199591971170104));
#3320=CARTESIAN_POINT('Ctrl Pts',(-1.10509821673782,-0.0928409665394228,
-0.204327142733962));
#3321=CARTESIAN_POINT('Ctrl Pts',(-1.10139388218929,-0.144299303100741,
-0.22376314604679));
#3322=CARTESIAN_POINT('Ctrl Pts',(-1.09728268713976,-0.177024326825049,
-0.243890930799338));
#3323=CARTESIAN_POINT('Ctrl Pts',(-1.08664560412098,-0.227269801620063,
-0.287406530683753));
#3324=CARTESIAN_POINT('Ctrl Pts',(-1.0788165083757,-0.251265615809407,-0.316022600643821));
#3325=CARTESIAN_POINT('Ctrl Pts',(-1.06356957703048,-0.279889827963178,
-0.363699428370918));
#3326=CARTESIAN_POINT('Ctrl Pts',(-1.05494634094458,-0.290879136862659,
-0.388295406390235));
#3327=CARTESIAN_POINT('Ctrl Pts',(-1.03504317708586,-0.305251990234488,
-0.438600874831839));
#3328=CARTESIAN_POINT('Ctrl Pts',(-1.02374168767024,-0.308638795020976,
-0.46430090015576));
#3329=CARTESIAN_POINT('Ctrl Pts',(-1.00129756308006,-0.308638795020976,
-0.510906605094603));
#3330=CARTESIAN_POINT('Ctrl Pts',(-0.988250837578047,-0.305251990234488,
-0.535766169015486));
#3331=CARTESIAN_POINT('Ctrl Pts',(-0.961329858300736,-0.290879136862659,
-0.582692035672022));
#3332=CARTESIAN_POINT('Ctrl Pts',(-0.947476448101718,-0.279889827963178,
-0.604769294586516));
#3333=CARTESIAN_POINT('Ctrl Pts',(-0.919707509403859,-0.251265615809407,
-0.646415841396062));
#3334=CARTESIAN_POINT('Ctrl Pts',(-0.902215926359523,-0.227269801620064,
-0.670378702718353));
#3335=CARTESIAN_POINT('Ctrl Pts',(-0.87482617317514,-0.177024326825049,
-0.705826641853758));
#3336=CARTESIAN_POINT('Ctrl Pts',(-0.861652925570091,-0.144299303100741,
-0.721590372101268));
#3337=CARTESIAN_POINT('Ctrl Pts',(-0.848766861100456,-0.0928409665394229,
-0.736604687327351));
#3338=CARTESIAN_POINT('Ctrl Pts',(-0.84559647055299,-0.0762225747374255,
-0.740223768851063));
#3339=CARTESIAN_POINT('Ctrl Pts',(-0.843383895613249,-0.0595300000000001,
-0.742736168477219));
#3340=CARTESIAN_POINT('',(-0.536443649899847,-0.05953,-0.987512846410683));
#3341=CARTESIAN_POINT('Origin',(0.,-0.05953,0.));
#3342=CARTESIAN_POINT('',(0.0548532617164172,-0.05953,-1.12247250791415));
#3343=CARTESIAN_POINT('Ctrl Pts',(-0.536443649899848,-0.0595300000000001,
-0.987512846410683));
#3344=CARTESIAN_POINT('Ctrl Pts',(-0.533501897135712,-0.0762225747374254,
-0.989110885965947));
#3345=CARTESIAN_POINT('Ctrl Pts',(-0.529268075276156,-0.0928409665394227,
-0.991396466802469));
#3346=CARTESIAN_POINT('Ctrl Pts',(-0.511762781179147,-0.144299303100741,
-1.00061845128527));
#3347=CARTESIAN_POINT('Ctrl Pts',(-0.493462957200432,-0.177024326825049,
-1.0099536580922));
#3348=CARTESIAN_POINT('Ctrl Pts',(-0.45280897844858,-0.227269801620063,
-1.02876878445619));
#3349=CARTESIAN_POINT('Ctrl Pts',(-0.425554672694337,-0.251265615809407,
-1.04048957871266));
#3350=CARTESIAN_POINT('Ctrl Pts',(-0.3787731215897,-0.279889827963178,-1.05829506364875));
#3351=CARTESIAN_POINT('Ctrl Pts',(-0.354166711873529,-0.290879136862659,
-1.06688848765783));
#3352=CARTESIAN_POINT('Ctrl Pts',(-0.302426893214944,-0.305251990234488,
-1.08269251410343));
#3353=CARTESIAN_POINT('Ctrl Pts',(-0.275287440920027,-0.308638795020976,
-1.0898803575765));
#3354=CARTESIAN_POINT('Ctrl Pts',(-0.224855950742601,-0.308638795020976,
-1.10139101611326));
#3355=CARTESIAN_POINT('Ctrl Pts',(-0.19728546073067,-0.305251990234488,
-1.10669035995599));
#3356=CARTESIAN_POINT('Ctrl Pts',(-0.143812384801039,-0.290879136862659,
-1.11490049012186));
#3357=CARTESIAN_POINT('Ctrl Pts',(-0.117914228755037,-0.279889827963178,
-1.1178344036749));
#3358=CARTESIAN_POINT('Ctrl Pts',(-0.0680399972366989,-0.251265615809407,
-1.12208997038458));
#3359=CARTESIAN_POINT('Ctrl Pts',(-0.0383992541984084,-0.227269801620063,
-1.12335509974011));
#3360=CARTESIAN_POINT('Ctrl Pts',(0.00639229239215326,-0.177024326825049,
-1.12404235695137));
#3361=CARTESIAN_POINT('Ctrl Pts',(0.0269302585198977,-0.144299303100741,
-1.12357162229597));
#3362=CARTESIAN_POINT('Ctrl Pts',(0.04670325263426,-0.0928409665394228,
-1.12285816383385));
#3363=CARTESIAN_POINT('Ctrl Pts',(0.0515094706813703,-0.0762225747374255,
-1.12263591311425));
#3364=CARTESIAN_POINT('Ctrl Pts',(0.0548532617164176,-0.0595300000000001,
-1.12247250791414));
#3365=CARTESIAN_POINT('',(0.437601487681057,-0.05953,-1.03511272300331));
#3366=CARTESIAN_POINT('Origin',(0.,-0.05953,0.));
#3367=CARTESIAN_POINT('',(0.911784794170997,-0.05953,-0.656964154625313));
#3368=CARTESIAN_POINT('Ctrl Pts',(0.437601487681056,-0.0595300000000001,
-1.03511272300331));
#3369=CARTESIAN_POINT('Ctrl Pts',(0.440685038163619,-0.0762225747374255,
-1.03380912944435));
#3370=CARTESIAN_POINT('Ctrl Pts',(0.445111721969657,-0.0928409665394228,
-1.03192403056628));
#3371=CARTESIAN_POINT('Ctrl Pts',(0.463236132117164,-0.144299303100741,
-1.0239876538093));
#3372=CARTESIAN_POINT('Ctrl Pts',(0.481944444320713,-0.177024326825049,
-1.01550068154148));
#3373=CARTESIAN_POINT('Ctrl Pts',(0.522002043615455,-0.227269801620064,
-0.995447160474328));
#3374=CARTESIAN_POINT('Ctrl Pts',(0.548158511259203,-0.251265615809407,
-0.981446681891443));
#3375=CARTESIAN_POINT('Ctrl Pts',(0.591247219971725,-0.279889827963178,
-0.955972930713954));
#3376=CARTESIAN_POINT('Ctrl Pts',(0.613307674922609,-0.290879136862659,
-0.942092777160053));
#3377=CARTESIAN_POINT('Ctrl Pts',(0.657923009631182,-0.305251990234487,
-0.91149460735272));
#3378=CARTESIAN_POINT('Ctrl Pts',(0.680463863683393,-0.308638795020976,
-0.894757676234429));
#3379=CARTESIAN_POINT('Ctrl Pts',(0.720906778729542,-0.308638795020976,
-0.862505527716294));
#3380=CARTESIAN_POINT('Ctrl Pts',(0.742239891936899,-0.305251990234488,
-0.844254137480381));
#3381=CARTESIAN_POINT('Ctrl Pts',(0.781998747691872,-0.290879136862659,
-0.80756613568454));
#3382=CARTESIAN_POINT('Ctrl Pts',(0.800439809856112,-0.279889827963178,
-0.789147407129765));
#3383=CARTESIAN_POINT('Ctrl Pts',(0.834863020612702,-0.251265615809407,
-0.752807465209441));
#3384=CARTESIAN_POINT('Ctrl Pts',(0.854332839576145,-0.227269801620064,
-0.73042219438957));
#3385=CARTESIAN_POINT('Ctrl Pts',(0.882797231409153,-0.177024326825049,
-0.695831250979106));
#3386=CARTESIAN_POINT('Ctrl Pts',(0.895234408667242,-0.144299303100741,
-0.679480524217551));
#3387=CARTESIAN_POINT('Ctrl Pts',(0.907004864562642,-0.0928409665394228,
-0.663576540841106));
#3388=CARTESIAN_POINT('Ctrl Pts',(0.909827729890942,-0.0762225747374256,
-0.659680317203144));
#3389=CARTESIAN_POINT('Ctrl Pts',(0.911784794170998,-0.0595300000000001,
-0.656964154625312));
#3390=CARTESIAN_POINT('',(1.08212377959455,-0.05953,-0.303251606722892));
#3391=CARTESIAN_POINT('Origin',(0.,-0.05953,0.));
#3392=CARTESIAN_POINT('',(1.08212377959455,-0.05953,0.303251606722892));
#3393=CARTESIAN_POINT('Ctrl Pts',(1.08212377959455,-0.0595300000000001,
-0.303251606722892));
#3394=CARTESIAN_POINT('Ctrl Pts',(1.0830271513892,-0.0762225747374255,-0.300028012588062));
#3395=CARTESIAN_POINT('Ctrl Pts',(1.08431331394788,-0.0928409665394228,
-0.2953917518996));
#3396=CARTESIAN_POINT('Ctrl Pts',(1.08940878963422,-0.144299303100741,-0.276273267473431));
#3397=CARTESIAN_POINT('Ctrl Pts',(1.09443784939331,-0.177024326825049,-0.256354979351213));
#3398=CARTESIAN_POINT('Ctrl Pts',(1.10373487993589,-0.227269801620064,-0.212533521233765));
#3399=CARTESIAN_POINT('Ctrl Pts',(1.10909715583869,-0.251265615809407,-0.183354415742157));
#3400=CARTESIAN_POINT('Ctrl Pts',(1.1160463456491,-0.279889827963178,-0.133783682657561));
#3401=CARTESIAN_POINT('Ctrl Pts',(1.11894887330541,-0.290879136862659,-0.107881990270302));
#3402=CARTESIAN_POINT('Ctrl Pts',(1.12284346704144,-0.305251990234488,-0.0539226701638766));
#3403=CARTESIAN_POINT('Ctrl Pts',(1.123812,-0.308638795020976,-0.025864214957475));
#3404=CARTESIAN_POINT('Ctrl Pts',(1.123812,-0.308638795020976,0.025864214957475));
#3405=CARTESIAN_POINT('Ctrl Pts',(1.12284346704144,-0.305251990234488,0.0539226701638766));
#3406=CARTESIAN_POINT('Ctrl Pts',(1.11894887330541,-0.290879136862659,0.107881990270302));
#3407=CARTESIAN_POINT('Ctrl Pts',(1.1160463456491,-0.279889827963178,0.133783682657561));
#3408=CARTESIAN_POINT('Ctrl Pts',(1.10909715583869,-0.251265615809407,0.183354415742157));
#3409=CARTESIAN_POINT('Ctrl Pts',(1.10373487993589,-0.227269801620064,0.212533521233765));
#3410=CARTESIAN_POINT('Ctrl Pts',(1.09443784939331,-0.177024326825049,0.256354979351213));
#3411=CARTESIAN_POINT('Ctrl Pts',(1.08940878963422,-0.144299303100741,0.276273267473431));
#3412=CARTESIAN_POINT('Ctrl Pts',(1.08431331394788,-0.0928409665394228,
0.2953917518996));
#3413=CARTESIAN_POINT('Ctrl Pts',(1.0830271513892,-0.0762225747374255,0.300028012588062));
#3414=CARTESIAN_POINT('Ctrl Pts',(1.08212377959455,-0.0595300000000001,
0.303251606722892));
#3415=CARTESIAN_POINT('Origin',(0.,-0.05953,0.));
#3416=CARTESIAN_POINT('Origin',(0.,-0.05953,0.));
#3417=CARTESIAN_POINT('',(0.0589974094846122,-0.05953,1.07456964270265));
#3418=CARTESIAN_POINT('Origin',(0.,-0.05953,0.));
#3419=CARTESIAN_POINT('Origin',(-0.244773027351946,-0.05953,1.07242070340001));
#3420=CARTESIAN_POINT('Origin',(-0.244773027351946,0.,1.07242070340001));
#3421=CARTESIAN_POINT('',(-0.519393123750572,-0.05953,0.942555777842682));
#3422=CARTESIAN_POINT('Ctrl Pts',(-0.519393123750572,-0.05953,0.942555777842682));
#3423=CARTESIAN_POINT('Ctrl Pts',(-0.513714466572041,-0.0925528133349865,
0.945684988399766));
#3424=CARTESIAN_POINT('Ctrl Pts',(-0.503136848051455,-0.124911173756694,
0.951483858396181));
#3425=CARTESIAN_POINT('Ctrl Pts',(-0.47593627990192,-0.177924977804098,
0.965323333309091));
#3426=CARTESIAN_POINT('Ctrl Pts',(-0.460931856495794,-0.199697230012983,
0.972669835243841));
#3427=CARTESIAN_POINT('Ctrl Pts',(-0.426157505475872,-0.237895043532788,
0.988400002689705));
#3428=CARTESIAN_POINT('Ctrl Pts',(-0.406380688682952,-0.254319232363049,
0.996771768218699));
#3429=CARTESIAN_POINT('Ctrl Pts',(-0.364750145543744,-0.28018331644634,
1.01272583306292));
#3430=CARTESIAN_POINT('Ctrl Pts',(-0.340838910881557,-0.29104845371857,
1.02112815447116));
#3431=CARTESIAN_POINT('Ctrl Pts',(-0.290495481564827,-0.30527573347708,
1.036574285215));
#3432=CARTESIAN_POINT('Ctrl Pts',(-0.264056468041074,-0.308638795020976,
1.04359501395068));
#3433=CARTESIAN_POINT('Ctrl Pts',(-0.214892249704082,-0.308638795020976,
1.05481642595959));
#3434=CARTESIAN_POINT('Ctrl Pts',(-0.188025341585962,-0.30527573347708,
1.05996242598502));
#3435=CARTESIAN_POINT('Ctrl Pts',(-0.135965654106109,-0.29104845371857,
1.06788913840721));
#3436=CARTESIAN_POINT('Ctrl Pts',(-0.110776745452494,-0.28018331644634,
1.07069360430242));
#3437=CARTESIAN_POINT('Ctrl Pts',(-0.0663467128214646,-0.254319232363049,
1.07438230428002));
#3438=CARTESIAN_POINT('Ctrl Pts',(-0.0448960436540983,-0.237895043532788,
1.07542044338697));
#3439=CARTESIAN_POINT('Ctrl Pts',(-0.00674037211528124,-0.199697230012983,
1.07633607767727));
#3440=CARTESIAN_POINT('Ctrl Pts',(0.00996567398334777,-0.177924977804098,
1.07622728347683));
#3441=CARTESIAN_POINT('Ctrl Pts',(0.0404772621979741,-0.124911173756694,
1.07556023164702));
#3442=CARTESIAN_POINT('Ctrl Pts',(0.0525234025782719,-0.0925528133349865,
1.07492508698591));
#3443=CARTESIAN_POINT('Ctrl Pts',(0.0589974094846124,-0.05953,1.07456964270265));
#3444=CARTESIAN_POINT('Origin',(-0.244773027351946,-0.05953,1.07242070340001));
#3445=CARTESIAN_POINT('Origin',(0.,-0.05953,0.));
#3446=CARTESIAN_POINT('',(-0.803348093619616,-0.05953,0.716109245731214));
#3447=CARTESIAN_POINT('Origin',(0.,-0.05953,0.));
#3448=CARTESIAN_POINT('Origin',(-0.991065754692661,-0.05953,0.477272113029314));
#3449=CARTESIAN_POINT('Origin',(-0.991065754692661,0.,0.477272113029314));
#3450=CARTESIAN_POINT('',(-1.06075609691358,-0.05953,0.181596019242328));
#3451=CARTESIAN_POINT('Ctrl Pts',(-1.06075609691358,-0.05953,0.181596019242328));
#3452=CARTESIAN_POINT('Ctrl Pts',(-1.05966202740332,-0.0925528133349865,
0.187986803072856));
#3453=CARTESIAN_POINT('Ctrl Pts',(-1.05760072925372,-0.124911173756694,
0.199872254546857));
#3454=CARTESIAN_POINT('Ctrl Pts',(-1.05146158959546,-0.177924977804098,
0.22976728653846));
#3455=CARTESIAN_POINT('Ctrl Pts',(-1.04785021111757,-0.199697230012983,
0.246078686169301));
#3456=CARTESIAN_POINT('Ctrl Pts',(-1.03846709802406,-0.237895043532788,
0.283073967563097));
#3457=CARTESIAN_POINT('Ctrl Pts',(-1.03268176429485,-0.254319232363049,
0.303755815985685));
#3458=CARTESIAN_POINT('Ctrl Pts',(-1.01919893537026,-0.28018331644634,0.346251081972725));
#3459=CARTESIAN_POINT('Ctrl Pts',(-1.01085972381132,-0.29104845371857,0.370184399726282));
#3460=CARTESIAN_POINT('Ctrl Pts',(-0.99154738033959,-0.30527573347708,0.419174982698463));
#3461=CARTESIAN_POINT('Ctrl Pts',(-0.980551951791748,-0.308638795020976,
0.444223188605045));
#3462=CARTESIAN_POINT('Ctrl Pts',(-0.958671816228589,-0.308638795020976,
0.489657758261848));
#3463=CARTESIAN_POINT('Ctrl Pts',(-0.945943877838127,-0.30527573347708,
0.51387163140139));
#3464=CARTESIAN_POINT('Ctrl Pts',(-0.91968254693063,-0.29104845371857,0.559515758398093));
#3465=CARTESIAN_POINT('Ctrl Pts',(-0.906170138993533,-0.28018331644634,
0.580957796077825));
#3466=CARTESIAN_POINT('Ctrl Pts',(-0.8813524085237,-0.254319232363049,0.617994461173994));
#3467=CARTESIAN_POINT('Ctrl Pts',(-0.868789784891799,-0.237895043532788,
0.635412538795143));
#3468=CARTESIAN_POINT('Ctrl Pts',(-0.845715984518854,-0.199697230012983,
0.66581473268113));
#3469=CARTESIAN_POINT('Ctrl Pts',(-0.835214876415962,-0.177924977804098,
0.678808213394124));
#3470=CARTESIAN_POINT('Ctrl Pts',(-0.815669690204649,-0.124911173756694,
0.702247233627224));
#3471=CARTESIAN_POINT('Ctrl Pts',(-0.807662468433796,-0.0925528133349865,
0.711269279199861));
#3472=CARTESIAN_POINT('Ctrl Pts',(-0.803348093619616,-0.05953,0.716109245731214));
#3473=CARTESIAN_POINT('Origin',(-0.991065754692661,-0.05953,0.477272113029314));
#3474=CARTESIAN_POINT('Origin',(0.,-0.05953,0.));
#3475=CARTESIAN_POINT('',(-1.076188,-0.05953,1.31795018948079E-16));
#3476=CARTESIAN_POINT('Origin',(0.,-0.05953,0.));
#3477=CARTESIAN_POINT('',(-1.06075609691358,-0.05953,-0.181596019242328));
#3478=CARTESIAN_POINT('Origin',(0.,-0.05953,0.));
#3479=CARTESIAN_POINT('Origin',(-0.991065754692661,-0.05953,-0.477272113029314));
#3480=CARTESIAN_POINT('Origin',(-0.991065754692661,0.,-0.477272113029314));
#3481=CARTESIAN_POINT('',(-0.803348093619616,-0.05953,-0.716109245731215));
#3482=CARTESIAN_POINT('Ctrl Pts',(-0.803348093619616,-0.05953,-0.716109245731215));
#3483=CARTESIAN_POINT('Ctrl Pts',(-0.807662468433795,-0.0925528133349865,
-0.711269279199862));
#3484=CARTESIAN_POINT('Ctrl Pts',(-0.815669690204649,-0.124911173756694,
-0.702247233627224));
#3485=CARTESIAN_POINT('Ctrl Pts',(-0.835214876415962,-0.177924977804098,
-0.678808213394124));
#3486=CARTESIAN_POINT('Ctrl Pts',(-0.845715984518854,-0.199697230012983,
-0.66581473268113));
#3487=CARTESIAN_POINT('Ctrl Pts',(-0.868789784891799,-0.237895043532788,
-0.635412538795143));
#3488=CARTESIAN_POINT('Ctrl Pts',(-0.8813524085237,-0.254319232363049,-0.617994461173994));
#3489=CARTESIAN_POINT('Ctrl Pts',(-0.906170138993533,-0.28018331644634,
-0.580957796077826));
#3490=CARTESIAN_POINT('Ctrl Pts',(-0.91968254693063,-0.29104845371857,-0.559515758398093));
#3491=CARTESIAN_POINT('Ctrl Pts',(-0.945943877838127,-0.30527573347708,
-0.51387163140139));
#3492=CARTESIAN_POINT('Ctrl Pts',(-0.958671816228589,-0.308638795020976,
-0.489657758261848));
#3493=CARTESIAN_POINT('Ctrl Pts',(-0.980551951791748,-0.308638795020976,
-0.444223188605045));
#3494=CARTESIAN_POINT('Ctrl Pts',(-0.99154738033959,-0.30527573347708,-0.419174982698463));
#3495=CARTESIAN_POINT('Ctrl Pts',(-1.01085972381132,-0.29104845371857,-0.370184399726282));
#3496=CARTESIAN_POINT('Ctrl Pts',(-1.01919893537026,-0.28018331644634,-0.346251081972725));
#3497=CARTESIAN_POINT('Ctrl Pts',(-1.03268176429485,-0.254319232363049,
-0.303755815985685));
#3498=CARTESIAN_POINT('Ctrl Pts',(-1.03846709802406,-0.237895043532788,
-0.283073967563097));
#3499=CARTESIAN_POINT('Ctrl Pts',(-1.04785021111757,-0.199697230012983,
-0.246078686169302));
#3500=CARTESIAN_POINT('Ctrl Pts',(-1.05146158959546,-0.177924977804098,
-0.229767286538461));
#3501=CARTESIAN_POINT('Ctrl Pts',(-1.05760072925372,-0.124911173756694,
-0.199872254546858));
#3502=CARTESIAN_POINT('Ctrl Pts',(-1.05966202740332,-0.0925528133349864,
-0.187986803072857));
#3503=CARTESIAN_POINT('Ctrl Pts',(-1.06075609691358,-0.05953,-0.181596019242328));
#3504=CARTESIAN_POINT('Origin',(-0.991065754692661,-0.05953,-0.477272113029314));
#3505=CARTESIAN_POINT('Origin',(0.,-0.05953,0.));
#3506=CARTESIAN_POINT('',(-0.519393123750572,-0.05953,-0.942555777842682));
#3507=CARTESIAN_POINT('Origin',(0.,-0.05953,0.));
#3508=CARTESIAN_POINT('Origin',(-0.244773027351946,-0.05953,-1.07242070340001));
#3509=CARTESIAN_POINT('Origin',(-0.244773027351946,0.,-1.07242070340001));
#3510=CARTESIAN_POINT('',(0.0589974094846125,-0.05953,-1.07456964270265));
#3511=CARTESIAN_POINT('Ctrl Pts',(0.0589974094846127,-0.05953,-1.07456964270265));
#3512=CARTESIAN_POINT('Ctrl Pts',(0.0525234025782722,-0.0925528133349865,
-1.07492508698591));
#3513=CARTESIAN_POINT('Ctrl Pts',(0.0404772621979744,-0.124911173756694,
-1.07556023164702));
#3514=CARTESIAN_POINT('Ctrl Pts',(0.0099656739833481,-0.177924977804098,
-1.07622728347683));
#3515=CARTESIAN_POINT('Ctrl Pts',(-0.00674037211528096,-0.199697230012983,
-1.07633607767727));
#3516=CARTESIAN_POINT('Ctrl Pts',(-0.044896043654098,-0.237895043532788,
-1.07542044338697));
#3517=CARTESIAN_POINT('Ctrl Pts',(-0.0663467128214644,-0.254319232363049,
-1.07438230428002));
#3518=CARTESIAN_POINT('Ctrl Pts',(-0.110776745452493,-0.28018331644634,
-1.07069360430242));
#3519=CARTESIAN_POINT('Ctrl Pts',(-0.135965654106109,-0.29104845371857,
-1.06788913840721));
#3520=CARTESIAN_POINT('Ctrl Pts',(-0.188025341585962,-0.30527573347708,
-1.05996242598502));
#3521=CARTESIAN_POINT('Ctrl Pts',(-0.214892249704082,-0.308638795020976,
-1.05481642595959));
#3522=CARTESIAN_POINT('Ctrl Pts',(-0.264056468041074,-0.308638795020976,
-1.04359501395068));
#3523=CARTESIAN_POINT('Ctrl Pts',(-0.290495481564827,-0.30527573347708,
-1.036574285215));
#3524=CARTESIAN_POINT('Ctrl Pts',(-0.340838910881557,-0.291048453718569,
-1.02112815447116));
#3525=CARTESIAN_POINT('Ctrl Pts',(-0.364750145543744,-0.28018331644634,
-1.01272583306292));
#3526=CARTESIAN_POINT('Ctrl Pts',(-0.406380688682952,-0.254319232363049,
-0.996771768218699));
#3527=CARTESIAN_POINT('Ctrl Pts',(-0.426157505475872,-0.237895043532788,
-0.988400002689705));
#3528=CARTESIAN_POINT('Ctrl Pts',(-0.460931856495794,-0.199697230012983,
-0.972669835243841));
#3529=CARTESIAN_POINT('Ctrl Pts',(-0.475936279901919,-0.177924977804098,
-0.965323333309091));
#3530=CARTESIAN_POINT('Ctrl Pts',(-0.503136848051454,-0.124911173756694,
-0.951483858396181));
#3531=CARTESIAN_POINT('Ctrl Pts',(-0.513714466572041,-0.0925528133349865,
-0.945684988399766));
#3532=CARTESIAN_POINT('Ctrl Pts',(-0.519393123750572,-0.05953,-0.942555777842682));
#3533=CARTESIAN_POINT('Origin',(-0.244773027351946,-0.05953,-1.07242070340001));
#3534=CARTESIAN_POINT('Origin',(0.,-0.05953,0.));
#3535=CARTESIAN_POINT('',(0.413083465285518,-0.05953,-0.993751811093549));
#3536=CARTESIAN_POINT('Origin',(0.,-0.05953,0.));
#3537=CARTESIAN_POINT('Origin',(0.685838782044607,-0.05953,-0.860014630714833));
#3538=CARTESIAN_POINT('Origin',(0.685838782044607,0.,-0.860014630714833));
#3539=CARTESIAN_POINT('',(0.876916659919095,-0.05953,-0.623857181492959));
#3540=CARTESIAN_POINT('Ctrl Pts',(0.876916659919095,-0.05953,-0.623857181492958));
#3541=CARTESIAN_POINT('Ctrl Pts',(0.873158080166742,-0.0925528133349865,
-0.62914037979579));
#3542=CARTESIAN_POINT('Ctrl Pts',(0.866144010579847,-0.124911173756694,
-0.638954437806245));
#3543=CARTESIAN_POINT('Ctrl Pts',(0.847641868610495,-0.177924977804098,
-0.663225258065736));
#3544=CARTESIAN_POINT('Ctrl Pts',(0.837310877969633,-0.199697230012983,
-0.676354402927683));
#3545=CARTESIAN_POINT('Ctrl Pts',(0.81280533416753,-0.237895043532788,-0.705614819529209));
#3546=CARTESIAN_POINT('Ctrl Pts',(0.798619410861634,-0.254319232363049,
-0.721738358858166));
#3547=CARTESIAN_POINT('Ctrl Pts',(0.768033796848072,-0.28018331644634,-0.754175290318038));
#3548=CARTESIAN_POINT('Ctrl Pts',(0.750136149454208,-0.29104845371857,-0.772120216227122));
#3549=CARTESIAN_POINT('Ctrl Pts',(0.711480111898423,-0.30527573347708,-0.807879894508811));
#3550=CARTESIAN_POINT('Ctrl Pts',(0.690705563850638,-0.308638795020976,
-0.825676810575913));
#3551=CARTESIAN_POINT('Ctrl Pts',(0.651278921914856,-0.308638795020976,
-0.857118508332695));
#3552=CARTESIAN_POINT('Ctrl Pts',(0.629305439856167,-0.30527573347708,-0.873412008702649));
#3553=CARTESIAN_POINT('Ctrl Pts',(0.585840553788742,-0.29104845371857,-0.903141581680914));
#3554=CARTESIAN_POINT('Ctrl Pts',(0.564362943424239,-0.28018331644634,-0.916597376014514));
#3555=CARTESIAN_POINT('Ctrl Pts',(0.525933334162556,-0.254319232363049,
-0.939198248544427));
#3556=CARTESIAN_POINT('Ctrl Pts',(0.507057380724533,-0.237895043532788,
-0.949440676105255));
#3557=CARTESIAN_POINT('Ctrl Pts',(0.473077587363686,-0.199697230012983,
-0.966820759530997));
#3558=CARTESIAN_POINT('Ctrl Pts',(0.457978755888596,-0.177924977804098,
-0.973971221090534));
#3559=CARTESIAN_POINT('Ctrl Pts',(0.430199341854858,-0.124911173756694,
-0.986608710139579));
#3560=CARTESIAN_POINT('Ctrl Pts',(0.419070565453384,-0.0925528133349865,
-0.991263089003441));
#3561=CARTESIAN_POINT('Ctrl Pts',(0.413083465285518,-0.05953,-0.993751811093549));
#3562=CARTESIAN_POINT('Origin',(0.685838782044607,-0.05953,-0.860014630714833));
#3563=CARTESIAN_POINT('Origin',(0.,-0.208355,0.));
#3564=CARTESIAN_POINT('',(-1.076188,-0.35718,1.31795018948079E-16));
#3565=CARTESIAN_POINT('Origin',(0.,-0.35718,0.));
#3566=CARTESIAN_POINT('',(-1.076188,-0.208355,1.31795018948079E-16));
#3567=CARTESIAN_POINT('',(1.03449977959455,-0.05953,0.296632461748266));
#3568=CARTESIAN_POINT('Origin',(0.,-0.05953,0.));
#3569=CARTESIAN_POINT('',(1.03449977959455,-0.05953,-0.296632461748266));
#3570=CARTESIAN_POINT('Ctrl Pts',(1.03449977959455,-0.05953,0.296632461748267));
#3571=CARTESIAN_POINT('Ctrl Pts',(1.03628691421076,-0.0925528133349865,
0.290399865505497));
#3572=CARTESIAN_POINT('Ctrl Pts',(1.03958665287714,-0.124911173756694,0.278797079997872));
#3573=CARTESIAN_POINT('Ctrl Pts',(1.0470264474309,-0.177924977804098,0.249198913998601));
#3574=CARTESIAN_POINT('Ctrl Pts',(1.05084995891418,-0.199697230012983,0.232935932341942));
#3575=CARTESIAN_POINT('Ctrl Pts',(1.05844771715377,-0.237895043532788,0.195533155353269));
#3576=CARTESIAN_POINT('Ctrl Pts',(1.06220882929878,-0.254319232363049,0.17438929156337));
#3577=CARTESIAN_POINT('Ctrl Pts',(1.06849922508772,-0.28018331644634,0.130252399648131));
#3578=CARTESIAN_POINT('Ctrl Pts',(1.07137013248666,-0.29104845371857,0.105070977154072));
#3579=CARTESIAN_POINT('Ctrl Pts',(1.07522652957392,-0.30527573347708,0.0525526752791107));
#3580=CARTESIAN_POINT('Ctrl Pts',(1.076188,-0.308638795020976,0.025214283908933));
#3581=CARTESIAN_POINT('Ctrl Pts',(1.076188,-0.308638795020976,-0.025214283908933));
#3582=CARTESIAN_POINT('Ctrl Pts',(1.07522652957392,-0.30527573347708,-0.0525526752791107));
#3583=CARTESIAN_POINT('Ctrl Pts',(1.07137013248666,-0.29104845371857,-0.105070977154072));
#3584=CARTESIAN_POINT('Ctrl Pts',(1.06849922508772,-0.28018331644634,-0.130252399648131));
#3585=CARTESIAN_POINT('Ctrl Pts',(1.06220882929878,-0.254319232363049,-0.17438929156337));
#3586=CARTESIAN_POINT('Ctrl Pts',(1.05844771715377,-0.237895043532788,-0.195533155353269));
#3587=CARTESIAN_POINT('Ctrl Pts',(1.05084995891418,-0.199697230012983,-0.232935932341942));
#3588=CARTESIAN_POINT('Ctrl Pts',(1.0470264474309,-0.177924977804098,-0.249198913998601));
#3589=CARTESIAN_POINT('Ctrl Pts',(1.03958665287714,-0.124911173756694,-0.278797079997872));
#3590=CARTESIAN_POINT('Ctrl Pts',(1.03628691421076,-0.0925528133349865,
-0.290399865505497));
#3591=CARTESIAN_POINT('Ctrl Pts',(1.03449977959455,-0.05953,-0.296632461748267));
#3592=CARTESIAN_POINT('Origin',(0.,-0.05953,0.));
#3593=CARTESIAN_POINT('Origin',(0.,-0.05953,0.));
#3594=CARTESIAN_POINT('Origin',(1.1,-0.05953,0.));
#3595=CARTESIAN_POINT('Origin',(1.1,0.,0.));
#3596=CARTESIAN_POINT('Origin',(1.1,-0.05953,0.));
#3597=CARTESIAN_POINT('Origin',(0.,-0.35718,0.));
#3598=CARTESIAN_POINT('Origin',(0.,-0.05953,0.));
#3668=UNCERTAINTY_MEASURE_WITH_UNIT(LENGTH_MEASURE(0.001),#3689,
'DISTANCE_ACCURACY_VALUE',
'Maximum model space distance between geometric entities at asserted c
onnectivities');
#3671=UNCERTAINTY_MEASURE_WITH_UNIT(LENGTH_MEASURE(0.001),#3689,
'DISTANCE_ACCURACY_VALUE',
'Maximum model space distance between geometric entities at asserted c
onnectivities');
#3685=(
GEOMETRIC_REPRESENTATION_CONTEXT(3)
GLOBAL_UNCERTAINTY_ASSIGNED_CONTEXT((#3668))
GLOBAL_UNIT_ASSIGNED_CONTEXT((#3689,#3691,#3692))
REPRESENTATION_CONTEXT('','3D')
);
#3688=(
GEOMETRIC_REPRESENTATION_CONTEXT(3)
GLOBAL_UNCERTAINTY_ASSIGNED_CONTEXT((#3671))
GLOBAL_UNIT_ASSIGNED_CONTEXT((#3689,#3691,#3692))
REPRESENTATION_CONTEXT('','3D')
);
#3689=(
LENGTH_UNIT()
NAMED_UNIT(*)
SI_UNIT(.CENTI.,.METRE.)
);
#3691=(
NAMED_UNIT(*)
PLANE_ANGLE_UNIT()
SI_UNIT($,.RADIAN.)
);
#3692=(
NAMED_UNIT(*)
SI_UNIT($,.STERADIAN.)
SOLID_ANGLE_UNIT()
);
#3706=SHAPE_DEFINITION_REPRESENTATION(#3728,#3756);
#3728=PRODUCT_DEFINITION_SHAPE('',$,#3773);
#3756=SHAPE_REPRESENTATION('',(#2133),#3685);
#3759=PRODUCT_DEFINITION_CONTEXT('part definition',#3809,'design');
#3773=PRODUCT_DEFINITION('Cage','Cage',#3789,#3759);
#3789=PRODUCT_DEFINITION_FORMATION('',$,#3824);
#3809=APPLICATION_CONTEXT(
'Core Data for Automotive Mechanical Design Process');
#3810=PRODUCT_CONTEXT('part definition',#3809,'mechanical');
#3824=PRODUCT('Cage','Cage','Cage',(#3810));
#3890=COLOUR_RGB('Grey',0.48,0.52,0.57);
#3891=FILL_AREA_STYLE_COLOUR('',#3890);
#3892=FILL_AREA_STYLE('',(#3891));
#3893=SURFACE_STYLE_FILL_AREA(#3892);
#3894=SURFACE_SIDE_STYLE('',(#3893));
#3895=SURFACE_STYLE_USAGE(.BOTH.,#3894);
#3896=PRESENTATION_STYLE_ASSIGNMENT((#3895));
ENDSEC;
END-ISO-10303-21;
